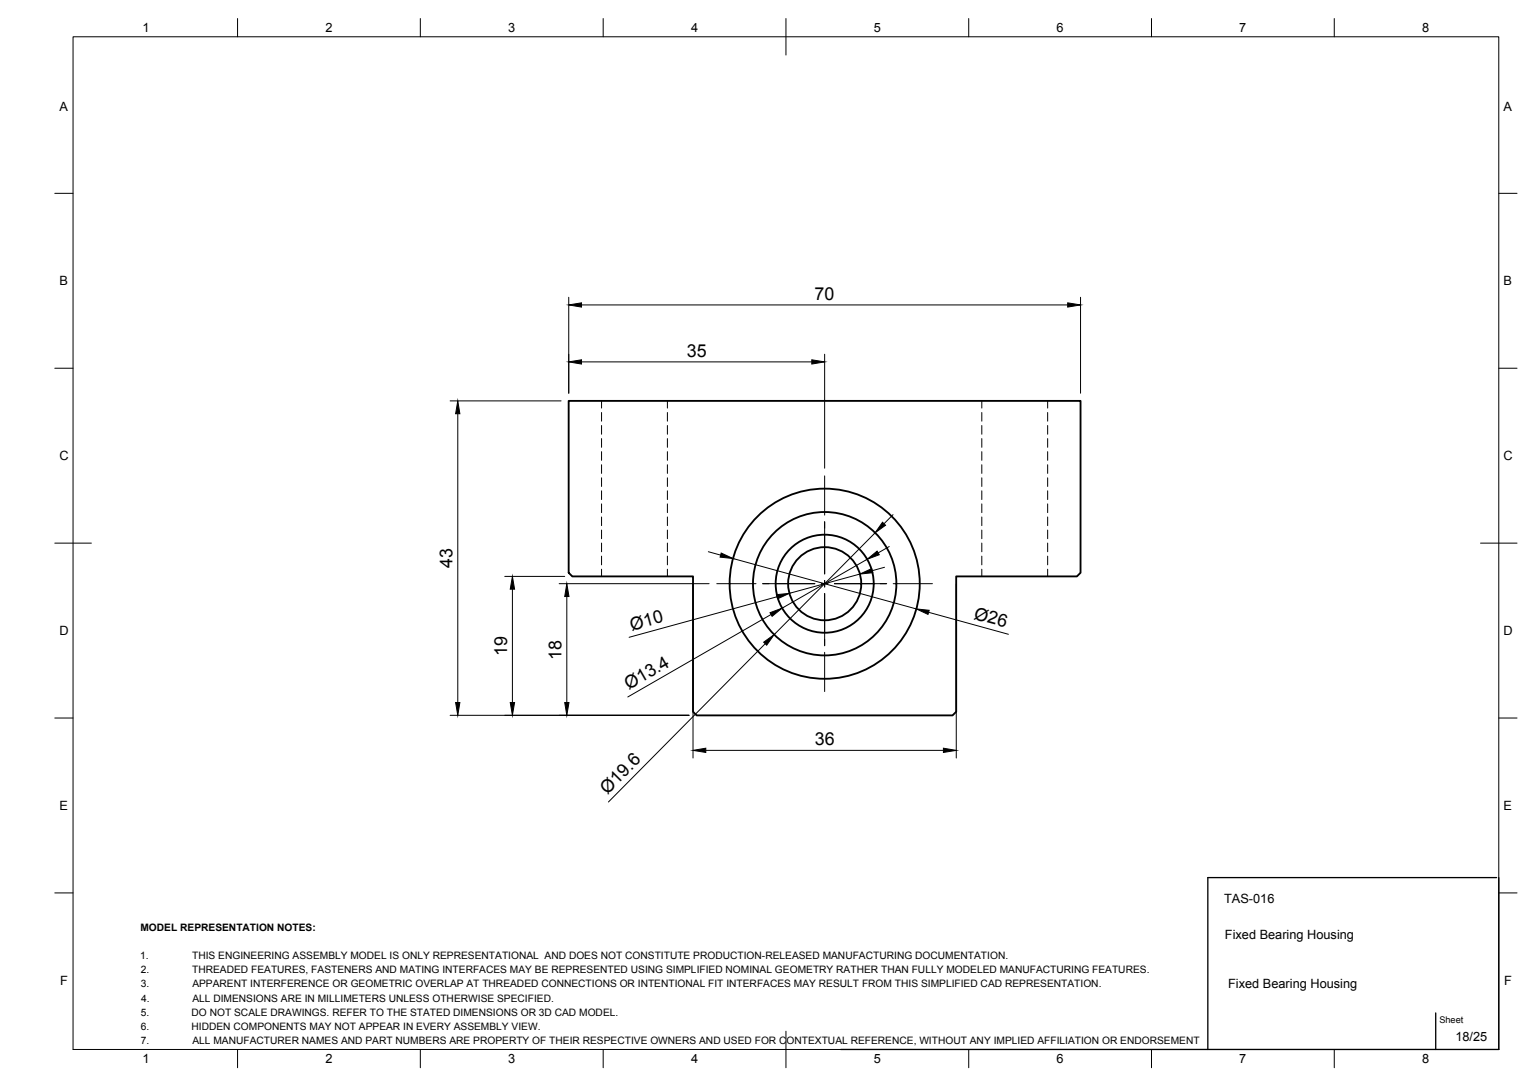
ISO-10303-21;
HEADER;
/* Generated by software containing ST-Developer
 * from STEP Tools, Inc. (www.steptools.com) 
 */

FILE_DESCRIPTION(
/* description */ ('STEP AP214'),
/* implementation_level */ '2;1');

FILE_NAME(
/* name */ 'Fixed Bearing Housing.step',
/* time_stamp */ '2026-11-15T14:55:55-08:00',
/* author */ (''),
/* organization */ (''),
/* preprocessor_version */ 'ST-DEVELOPER v20.2',
/* originating_system */ 'Autodesk Translation Framework v15.17.0.0',
/* authorisation */ '');

FILE_SCHEMA (('AUTOMOTIVE_DESIGN { 1 0 10303 214 3 1 1 }'));
ENDSEC;

DATA;
#10=MECHANICAL_DESIGN_GEOMETRIC_PRESENTATION_REPRESENTATION('',(#933,#934),#57079);
#644=TOROIDAL_SURFACE('',#25301,5.3,0.300000000000002);
#645=TOROIDAL_SURFACE('',#25307,5.3,0.300000000000002);
#646=TOROIDAL_SURFACE('',#25316,12.7,0.300000000000001);
#647=TOROIDAL_SURFACE('',#25322,12.7,0.300000000000002);
#874=SHAPE_REPRESENTATION_RELATIONSHIP('SRR','None',#57260,#903);
#903=ADVANCED_BREP_SHAPE_REPRESENTATION('',(#970,#971),#57052);
#933=STYLED_ITEM('',(#57444),#970);
#934=STYLED_ITEM('',(#57444),#971);
#970=MANIFOLD_SOLID_BREP('Body1',#24533);
#971=MANIFOLD_SOLID_BREP('Body2',#24534);
#1077=FACE_BOUND('',#3829,.T.);
#1078=FACE_BOUND('',#3831,.T.);
#1079=FACE_BOUND('',#3833,.T.);
#1080=FACE_BOUND('',#3837,.T.);
#1081=FACE_BOUND('',#3838,.T.);
#1082=FACE_BOUND('',#3842,.T.);
#1083=FACE_BOUND('',#3859,.T.);
#1084=FACE_BOUND('',#3861,.T.);
#1085=FACE_BOUND('',#3863,.T.);
#1086=FACE_BOUND('',#3865,.T.);
#1087=FACE_BOUND('',#3867,.T.);
#1088=FACE_BOUND('',#3869,.T.);
#1472=PLANE('',#25287);
#1473=PLANE('',#25288);
#1474=PLANE('',#25289);
#1475=PLANE('',#25290);
#1476=PLANE('',#25291);
#1477=PLANE('',#25292);
#1478=PLANE('',#25293);
#1479=PLANE('',#25294);
#1480=PLANE('',#25295);
#1481=PLANE('',#25296);
#1482=PLANE('',#25297);
#1483=PLANE('',#25298);
#1484=PLANE('',#25299);
#1485=PLANE('',#25300);
#1486=PLANE('',#25331);
#1487=PLANE('',#25332);
#1488=PLANE('',#25333);
#1489=PLANE('',#25334);
#1490=PLANE('',#25335);
#1491=PLANE('',#25336);
#2373=FACE_OUTER_BOUND('',#3825,.T.);
#2374=FACE_OUTER_BOUND('',#3826,.T.);
#2375=FACE_OUTER_BOUND('',#3827,.T.);
#2376=FACE_OUTER_BOUND('',#3828,.T.);
#2377=FACE_OUTER_BOUND('',#3830,.T.);
#2378=FACE_OUTER_BOUND('',#3832,.T.);
#2379=FACE_OUTER_BOUND('',#3834,.T.);
#2380=FACE_OUTER_BOUND('',#3835,.T.);
#2381=FACE_OUTER_BOUND('',#3836,.T.);
#2382=FACE_OUTER_BOUND('',#3839,.T.);
#2383=FACE_OUTER_BOUND('',#3840,.T.);
#2384=FACE_OUTER_BOUND('',#3841,.T.);
#2385=FACE_OUTER_BOUND('',#3843,.T.);
#2386=FACE_OUTER_BOUND('',#3844,.T.);
#2387=FACE_OUTER_BOUND('',#3845,.T.);
#2388=FACE_OUTER_BOUND('',#3846,.T.);
#2389=FACE_OUTER_BOUND('',#3847,.T.);
#2390=FACE_OUTER_BOUND('',#3848,.T.);
#2391=FACE_OUTER_BOUND('',#3849,.T.);
#2392=FACE_OUTER_BOUND('',#3850,.T.);
#2393=FACE_OUTER_BOUND('',#3851,.T.);
#2394=FACE_OUTER_BOUND('',#3852,.T.);
#2395=FACE_OUTER_BOUND('',#3853,.T.);
#2396=FACE_OUTER_BOUND('',#3854,.T.);
#2397=FACE_OUTER_BOUND('',#3855,.T.);
#2398=FACE_OUTER_BOUND('',#3856,.T.);
#2399=FACE_OUTER_BOUND('',#3857,.T.);
#2400=FACE_OUTER_BOUND('',#3858,.T.);
#2401=FACE_OUTER_BOUND('',#3860,.T.);
#2402=FACE_OUTER_BOUND('',#3862,.T.);
#2403=FACE_OUTER_BOUND('',#3864,.T.);
#2404=FACE_OUTER_BOUND('',#3866,.T.);
#2405=FACE_OUTER_BOUND('',#3868,.T.);
#3825=EDGE_LOOP('',(#16870,#16871,#16872,#16873));
#3826=EDGE_LOOP('',(#16874,#16875,#16876,#16877));
#3827=EDGE_LOOP('',(#16878,#16879,#16880,#16881));
#3828=EDGE_LOOP('',(#16882,#16883,#16884,#16885,#16886,#16887,#16888,#16889,
#16890,#16891,#16892,#16893));
#3829=EDGE_LOOP('',(#16894));
#3830=EDGE_LOOP('',(#16895,#16896,#16897,#16898,#16899,#16900,#16901,#16902,
#16903,#16904,#16905,#16906));
#3831=EDGE_LOOP('',(#16907));
#3832=EDGE_LOOP('',(#16908,#16909,#16910,#16911));
#3833=EDGE_LOOP('',(#16912));
#3834=EDGE_LOOP('',(#16913,#16914,#16915,#16916));
#3835=EDGE_LOOP('',(#16917,#16918,#16919,#16920));
#3836=EDGE_LOOP('',(#16921,#16922,#16923,#16924));
#3837=EDGE_LOOP('',(#16925));
#3838=EDGE_LOOP('',(#16926));
#3839=EDGE_LOOP('',(#16927,#16928,#16929,#16930));
#3840=EDGE_LOOP('',(#16931,#16932,#16933,#16934));
#3841=EDGE_LOOP('',(#16935,#16936,#16937,#16938));
#3842=EDGE_LOOP('',(#16939));
#3843=EDGE_LOOP('',(#16940,#16941,#16942,#16943));
#3844=EDGE_LOOP('',(#16944,#16945,#16946,#16947));
#3845=EDGE_LOOP('',(#16948,#16949,#16950,#16951));
#3846=EDGE_LOOP('',(#16952,#16953,#16954,#16955));
#3847=EDGE_LOOP('',(#16956,#16957,#16958,#16959));
#3848=EDGE_LOOP('',(#16960,#16961,#16962,#16963));
#3849=EDGE_LOOP('',(#16964,#16965,#16966,#16967));
#3850=EDGE_LOOP('',(#16968,#16969,#16970,#16971));
#3851=EDGE_LOOP('',(#16972,#16973,#16974,#16975));
#3852=EDGE_LOOP('',(#16976,#16977,#16978,#16979));
#3853=EDGE_LOOP('',(#16980,#16981,#16982,#16983));
#3854=EDGE_LOOP('',(#16984,#16985,#16986,#16987));
#3855=EDGE_LOOP('',(#16988,#16989,#16990,#16991));
#3856=EDGE_LOOP('',(#16992,#16993,#16994,#16995));
#3857=EDGE_LOOP('',(#16996,#16997,#16998,#16999));
#3858=EDGE_LOOP('',(#17000));
#3859=EDGE_LOOP('',(#17001));
#3860=EDGE_LOOP('',(#17002));
#3861=EDGE_LOOP('',(#17003));
#3862=EDGE_LOOP('',(#17004));
#3863=EDGE_LOOP('',(#17005));
#3864=EDGE_LOOP('',(#17006));
#3865=EDGE_LOOP('',(#17007));
#3866=EDGE_LOOP('',(#17008));
#3867=EDGE_LOOP('',(#17009));
#3868=EDGE_LOOP('',(#17010));
#3869=EDGE_LOOP('',(#17011));
#5550=LINE('',#35882,#7517);
#5551=LINE('',#35888,#7518);
#5552=LINE('',#35894,#7519);
#5553=LINE('',#35899,#7520);
#5554=LINE('',#35901,#7521);
#5555=LINE('',#35903,#7522);
#5556=LINE('',#35905,#7523);
#5557=LINE('',#35907,#7524);
#5558=LINE('',#35909,#7525);
#5559=LINE('',#35911,#7526);
#5560=LINE('',#35913,#7527);
#5561=LINE('',#35915,#7528);
#5562=LINE('',#35917,#7529);
#5563=LINE('',#35919,#7530);
#5564=LINE('',#35920,#7531);
#5565=LINE('',#35924,#7532);
#5566=LINE('',#35926,#7533);
#5567=LINE('',#35928,#7534);
#5568=LINE('',#35930,#7535);
#5569=LINE('',#35932,#7536);
#5570=LINE('',#35934,#7537);
#5571=LINE('',#35936,#7538);
#5572=LINE('',#35938,#7539);
#5573=LINE('',#35940,#7540);
#5574=LINE('',#35942,#7541);
#5575=LINE('',#35944,#7542);
#5576=LINE('',#35945,#7543);
#5577=LINE('',#35947,#7544);
#5578=LINE('',#35948,#7545);
#5579=LINE('',#35950,#7546);
#5580=LINE('',#35952,#7547);
#5581=LINE('',#35954,#7548);
#5582=LINE('',#35956,#7549);
#5583=LINE('',#35958,#7550);
#5584=LINE('',#35960,#7551);
#5585=LINE('',#35962,#7552);
#5586=LINE('',#35964,#7553);
#5587=LINE('',#35966,#7554);
#5588=LINE('',#35968,#7555);
#5589=LINE('',#35978,#7556);
#5590=LINE('',#35988,#7557);
#5591=LINE('',#35994,#7558);
#5592=LINE('',#36004,#7559);
#5593=LINE('',#36014,#7560);
#5594=LINE('',#36020,#7561);
#7517=VECTOR('',#28570,4.49999999999999);
#7518=VECTOR('',#28577,4.49999999999999);
#7519=VECTOR('',#28584,13.);
#7520=VECTOR('',#28589,1000.);
#7521=VECTOR('',#28590,1000.);
#7522=VECTOR('',#28591,1000.);
#7523=VECTOR('',#28592,1000.);
#7524=VECTOR('',#28593,1000.);
#7525=VECTOR('',#28594,1000.);
#7526=VECTOR('',#28595,1000.);
#7527=VECTOR('',#28596,1000.);
#7528=VECTOR('',#28597,1000.);
#7529=VECTOR('',#28598,1000.);
#7530=VECTOR('',#28599,1000.);
#7531=VECTOR('',#28600,1000.);
#7532=VECTOR('',#28603,1000.);
#7533=VECTOR('',#28604,1000.);
#7534=VECTOR('',#28605,1000.);
#7535=VECTOR('',#28606,1000.);
#7536=VECTOR('',#28607,1000.);
#7537=VECTOR('',#28608,1000.);
#7538=VECTOR('',#28609,1000.);
#7539=VECTOR('',#28610,1000.);
#7540=VECTOR('',#28611,1000.);
#7541=VECTOR('',#28612,1000.);
#7542=VECTOR('',#28613,1000.);
#7543=VECTOR('',#28614,1000.);
#7544=VECTOR('',#28617,1000.);
#7545=VECTOR('',#28618,1000.);
#7546=VECTOR('',#28621,1000.);
#7547=VECTOR('',#28624,1000.);
#7548=VECTOR('',#28627,1000.);
#7549=VECTOR('',#28630,1000.);
#7550=VECTOR('',#28633,1000.);
#7551=VECTOR('',#28636,1000.);
#7552=VECTOR('',#28639,1000.);
#7553=VECTOR('',#28642,1000.);
#7554=VECTOR('',#28645,1000.);
#7555=VECTOR('',#28648,1000.);
#7556=VECTOR('',#28661,5.);
#7557=VECTOR('',#28674,6.7);
#7558=VECTOR('',#28681,9.8);
#7559=VECTOR('',#28694,13.);
#7560=VECTOR('',#28707,9.8);
#7561=VECTOR('',#28714,6.69999999999999);
#9348=CIRCLE('',#25279,4.5);
#9349=CIRCLE('',#25280,4.49999999999999);
#9350=CIRCLE('',#25282,4.5);
#9351=CIRCLE('',#25283,4.49999999999999);
#9352=CIRCLE('',#25285,13.);
#9353=CIRCLE('',#25286,13.);
#9354=CIRCLE('',#25302,5.3);
#9355=CIRCLE('',#25303,0.300000000000002);
#9356=CIRCLE('',#25304,4.99999999999999);
#9357=CIRCLE('',#25306,5.);
#9358=CIRCLE('',#25308,0.300000000000002);
#9359=CIRCLE('',#25309,5.3);
#9360=CIRCLE('',#25311,6.7);
#9361=CIRCLE('',#25312,6.7);
#9362=CIRCLE('',#25314,9.8);
#9363=CIRCLE('',#25315,9.8);
#9364=CIRCLE('',#25317,12.7);
#9365=CIRCLE('',#25318,0.300000000000001);
#9366=CIRCLE('',#25319,13.);
#9367=CIRCLE('',#25321,13.);
#9368=CIRCLE('',#25323,0.300000000000002);
#9369=CIRCLE('',#25324,12.7);
#9370=CIRCLE('',#25326,9.8);
#9371=CIRCLE('',#25327,9.8);
#9372=CIRCLE('',#25329,6.69999999999999);
#9373=CIRCLE('',#25330,6.69999999999999);
#10589=VERTEX_POINT('',#35879);
#10590=VERTEX_POINT('',#35881);
#10591=VERTEX_POINT('',#35885);
#10592=VERTEX_POINT('',#35887);
#10593=VERTEX_POINT('',#35891);
#10594=VERTEX_POINT('',#35893);
#10595=VERTEX_POINT('',#35897);
#10596=VERTEX_POINT('',#35898);
#10597=VERTEX_POINT('',#35900);
#10598=VERTEX_POINT('',#35902);
#10599=VERTEX_POINT('',#35904);
#10600=VERTEX_POINT('',#35906);
#10601=VERTEX_POINT('',#35908);
#10602=VERTEX_POINT('',#35910);
#10603=VERTEX_POINT('',#35912);
#10604=VERTEX_POINT('',#35914);
#10605=VERTEX_POINT('',#35916);
#10606=VERTEX_POINT('',#35918);
#10607=VERTEX_POINT('',#35922);
#10608=VERTEX_POINT('',#35923);
#10609=VERTEX_POINT('',#35925);
#10610=VERTEX_POINT('',#35927);
#10611=VERTEX_POINT('',#35929);
#10612=VERTEX_POINT('',#35931);
#10613=VERTEX_POINT('',#35933);
#10614=VERTEX_POINT('',#35935);
#10615=VERTEX_POINT('',#35937);
#10616=VERTEX_POINT('',#35939);
#10617=VERTEX_POINT('',#35941);
#10618=VERTEX_POINT('',#35943);
#10619=VERTEX_POINT('',#35971);
#10620=VERTEX_POINT('',#35973);
#10621=VERTEX_POINT('',#35977);
#10622=VERTEX_POINT('',#35981);
#10623=VERTEX_POINT('',#35985);
#10624=VERTEX_POINT('',#35987);
#10625=VERTEX_POINT('',#35991);
#10626=VERTEX_POINT('',#35993);
#10627=VERTEX_POINT('',#35997);
#10628=VERTEX_POINT('',#35999);
#10629=VERTEX_POINT('',#36003);
#10630=VERTEX_POINT('',#36007);
#10631=VERTEX_POINT('',#36011);
#10632=VERTEX_POINT('',#36013);
#10633=VERTEX_POINT('',#36017);
#10634=VERTEX_POINT('',#36019);
#12980=EDGE_CURVE('',#10589,#10589,#9348,.T.);
#12981=EDGE_CURVE('',#10589,#10590,#5550,.T.);
#12982=EDGE_CURVE('',#10590,#10590,#9349,.T.);
#12983=EDGE_CURVE('',#10591,#10591,#9350,.T.);
#12984=EDGE_CURVE('',#10591,#10592,#5551,.T.);
#12985=EDGE_CURVE('',#10592,#10592,#9351,.T.);
#12986=EDGE_CURVE('',#10593,#10593,#9352,.T.);
#12987=EDGE_CURVE('',#10593,#10594,#5552,.T.);
#12988=EDGE_CURVE('',#10594,#10594,#9353,.T.);
#12989=EDGE_CURVE('',#10595,#10596,#5553,.T.);
#12990=EDGE_CURVE('',#10596,#10597,#5554,.T.);
#12991=EDGE_CURVE('',#10597,#10598,#5555,.T.);
#12992=EDGE_CURVE('',#10598,#10599,#5556,.T.);
#12993=EDGE_CURVE('',#10599,#10600,#5557,.T.);
#12994=EDGE_CURVE('',#10600,#10601,#5558,.T.);
#12995=EDGE_CURVE('',#10601,#10602,#5559,.T.);
#12996=EDGE_CURVE('',#10602,#10603,#5560,.T.);
#12997=EDGE_CURVE('',#10603,#10604,#5561,.T.);
#12998=EDGE_CURVE('',#10604,#10605,#5562,.T.);
#12999=EDGE_CURVE('',#10605,#10606,#5563,.T.);
#13000=EDGE_CURVE('',#10606,#10595,#5564,.T.);
#13001=EDGE_CURVE('',#10607,#10608,#5565,.T.);
#13002=EDGE_CURVE('',#10609,#10607,#5566,.T.);
#13003=EDGE_CURVE('',#10610,#10609,#5567,.T.);
#13004=EDGE_CURVE('',#10611,#10610,#5568,.T.);
#13005=EDGE_CURVE('',#10612,#10611,#5569,.T.);
#13006=EDGE_CURVE('',#10613,#10612,#5570,.T.);
#13007=EDGE_CURVE('',#10614,#10613,#5571,.T.);
#13008=EDGE_CURVE('',#10615,#10614,#5572,.T.);
#13009=EDGE_CURVE('',#10616,#10615,#5573,.T.);
#13010=EDGE_CURVE('',#10617,#10616,#5574,.T.);
#13011=EDGE_CURVE('',#10618,#10617,#5575,.T.);
#13012=EDGE_CURVE('',#10608,#10618,#5576,.T.);
#13013=EDGE_CURVE('',#10596,#10608,#5577,.T.);
#13014=EDGE_CURVE('',#10595,#10607,#5578,.T.);
#13015=EDGE_CURVE('',#10597,#10618,#5579,.T.);
#13016=EDGE_CURVE('',#10598,#10617,#5580,.T.);
#13017=EDGE_CURVE('',#10599,#10616,#5581,.T.);
#13018=EDGE_CURVE('',#10600,#10615,#5582,.T.);
#13019=EDGE_CURVE('',#10601,#10614,#5583,.T.);
#13020=EDGE_CURVE('',#10602,#10613,#5584,.T.);
#13021=EDGE_CURVE('',#10603,#10612,#5585,.T.);
#13022=EDGE_CURVE('',#10604,#10611,#5586,.T.);
#13023=EDGE_CURVE('',#10605,#10610,#5587,.T.);
#13024=EDGE_CURVE('',#10606,#10609,#5588,.T.);
#13025=EDGE_CURVE('',#10619,#10619,#9354,.T.);
#13026=EDGE_CURVE('',#10619,#10620,#9355,.T.);
#13027=EDGE_CURVE('',#10620,#10620,#9356,.T.);
#13028=EDGE_CURVE('',#10620,#10621,#5589,.T.);
#13029=EDGE_CURVE('',#10621,#10621,#9357,.T.);
#13030=EDGE_CURVE('',#10621,#10622,#9358,.T.);
#13031=EDGE_CURVE('',#10622,#10622,#9359,.T.);
#13032=EDGE_CURVE('',#10623,#10623,#9360,.T.);
#13033=EDGE_CURVE('',#10623,#10624,#5590,.T.);
#13034=EDGE_CURVE('',#10624,#10624,#9361,.T.);
#13035=EDGE_CURVE('',#10625,#10625,#9362,.T.);
#13036=EDGE_CURVE('',#10625,#10626,#5591,.T.);
#13037=EDGE_CURVE('',#10626,#10626,#9363,.T.);
#13038=EDGE_CURVE('',#10627,#10627,#9364,.T.);
#13039=EDGE_CURVE('',#10627,#10628,#9365,.T.);
#13040=EDGE_CURVE('',#10628,#10628,#9366,.T.);
#13041=EDGE_CURVE('',#10628,#10629,#5592,.T.);
#13042=EDGE_CURVE('',#10629,#10629,#9367,.T.);
#13043=EDGE_CURVE('',#10629,#10630,#9368,.T.);
#13044=EDGE_CURVE('',#10630,#10630,#9369,.T.);
#13045=EDGE_CURVE('',#10631,#10631,#9370,.T.);
#13046=EDGE_CURVE('',#10631,#10632,#5593,.T.);
#13047=EDGE_CURVE('',#10632,#10632,#9371,.T.);
#13048=EDGE_CURVE('',#10633,#10633,#9372,.T.);
#13049=EDGE_CURVE('',#10633,#10634,#5594,.T.);
#13050=EDGE_CURVE('',#10634,#10634,#9373,.T.);
#16870=ORIENTED_EDGE('',*,*,#12980,.F.);
#16871=ORIENTED_EDGE('',*,*,#12981,.T.);
#16872=ORIENTED_EDGE('',*,*,#12982,.T.);
#16873=ORIENTED_EDGE('',*,*,#12981,.F.);
#16874=ORIENTED_EDGE('',*,*,#12983,.F.);
#16875=ORIENTED_EDGE('',*,*,#12984,.T.);
#16876=ORIENTED_EDGE('',*,*,#12985,.T.);
#16877=ORIENTED_EDGE('',*,*,#12984,.F.);
#16878=ORIENTED_EDGE('',*,*,#12986,.T.);
#16879=ORIENTED_EDGE('',*,*,#12987,.T.);
#16880=ORIENTED_EDGE('',*,*,#12988,.F.);
#16881=ORIENTED_EDGE('',*,*,#12987,.F.);
#16882=ORIENTED_EDGE('',*,*,#12989,.T.);
#16883=ORIENTED_EDGE('',*,*,#12990,.T.);
#16884=ORIENTED_EDGE('',*,*,#12991,.T.);
#16885=ORIENTED_EDGE('',*,*,#12992,.T.);
#16886=ORIENTED_EDGE('',*,*,#12993,.T.);
#16887=ORIENTED_EDGE('',*,*,#12994,.T.);
#16888=ORIENTED_EDGE('',*,*,#12995,.T.);
#16889=ORIENTED_EDGE('',*,*,#12996,.T.);
#16890=ORIENTED_EDGE('',*,*,#12997,.T.);
#16891=ORIENTED_EDGE('',*,*,#12998,.T.);
#16892=ORIENTED_EDGE('',*,*,#12999,.T.);
#16893=ORIENTED_EDGE('',*,*,#13000,.T.);
#16894=ORIENTED_EDGE('',*,*,#12986,.F.);
#16895=ORIENTED_EDGE('',*,*,#13001,.F.);
#16896=ORIENTED_EDGE('',*,*,#13002,.F.);
#16897=ORIENTED_EDGE('',*,*,#13003,.F.);
#16898=ORIENTED_EDGE('',*,*,#13004,.F.);
#16899=ORIENTED_EDGE('',*,*,#13005,.F.);
#16900=ORIENTED_EDGE('',*,*,#13006,.F.);
#16901=ORIENTED_EDGE('',*,*,#13007,.F.);
#16902=ORIENTED_EDGE('',*,*,#13008,.F.);
#16903=ORIENTED_EDGE('',*,*,#13009,.F.);
#16904=ORIENTED_EDGE('',*,*,#13010,.F.);
#16905=ORIENTED_EDGE('',*,*,#13011,.F.);
#16906=ORIENTED_EDGE('',*,*,#13012,.F.);
#16907=ORIENTED_EDGE('',*,*,#12988,.T.);
#16908=ORIENTED_EDGE('',*,*,#13001,.T.);
#16909=ORIENTED_EDGE('',*,*,#13013,.F.);
#16910=ORIENTED_EDGE('',*,*,#12989,.F.);
#16911=ORIENTED_EDGE('',*,*,#13014,.T.);
#16912=ORIENTED_EDGE('',*,*,#12982,.F.);
#16913=ORIENTED_EDGE('',*,*,#13012,.T.);
#16914=ORIENTED_EDGE('',*,*,#13015,.F.);
#16915=ORIENTED_EDGE('',*,*,#12990,.F.);
#16916=ORIENTED_EDGE('',*,*,#13013,.T.);
#16917=ORIENTED_EDGE('',*,*,#13011,.T.);
#16918=ORIENTED_EDGE('',*,*,#13016,.F.);
#16919=ORIENTED_EDGE('',*,*,#12991,.F.);
#16920=ORIENTED_EDGE('',*,*,#13015,.T.);
#16921=ORIENTED_EDGE('',*,*,#13010,.T.);
#16922=ORIENTED_EDGE('',*,*,#13017,.F.);
#16923=ORIENTED_EDGE('',*,*,#12992,.F.);
#16924=ORIENTED_EDGE('',*,*,#13016,.T.);
#16925=ORIENTED_EDGE('',*,*,#12980,.T.);
#16926=ORIENTED_EDGE('',*,*,#12983,.T.);
#16927=ORIENTED_EDGE('',*,*,#13009,.T.);
#16928=ORIENTED_EDGE('',*,*,#13018,.F.);
#16929=ORIENTED_EDGE('',*,*,#12993,.F.);
#16930=ORIENTED_EDGE('',*,*,#13017,.T.);
#16931=ORIENTED_EDGE('',*,*,#13008,.T.);
#16932=ORIENTED_EDGE('',*,*,#13019,.F.);
#16933=ORIENTED_EDGE('',*,*,#12994,.F.);
#16934=ORIENTED_EDGE('',*,*,#13018,.T.);
#16935=ORIENTED_EDGE('',*,*,#13007,.T.);
#16936=ORIENTED_EDGE('',*,*,#13020,.F.);
#16937=ORIENTED_EDGE('',*,*,#12995,.F.);
#16938=ORIENTED_EDGE('',*,*,#13019,.T.);
#16939=ORIENTED_EDGE('',*,*,#12985,.F.);
#16940=ORIENTED_EDGE('',*,*,#13006,.T.);
#16941=ORIENTED_EDGE('',*,*,#13021,.F.);
#16942=ORIENTED_EDGE('',*,*,#12996,.F.);
#16943=ORIENTED_EDGE('',*,*,#13020,.T.);
#16944=ORIENTED_EDGE('',*,*,#13005,.T.);
#16945=ORIENTED_EDGE('',*,*,#13022,.F.);
#16946=ORIENTED_EDGE('',*,*,#12997,.F.);
#16947=ORIENTED_EDGE('',*,*,#13021,.T.);
#16948=ORIENTED_EDGE('',*,*,#13004,.T.);
#16949=ORIENTED_EDGE('',*,*,#13023,.F.);
#16950=ORIENTED_EDGE('',*,*,#12998,.F.);
#16951=ORIENTED_EDGE('',*,*,#13022,.T.);
#16952=ORIENTED_EDGE('',*,*,#13003,.T.);
#16953=ORIENTED_EDGE('',*,*,#13024,.F.);
#16954=ORIENTED_EDGE('',*,*,#12999,.F.);
#16955=ORIENTED_EDGE('',*,*,#13023,.T.);
#16956=ORIENTED_EDGE('',*,*,#13002,.T.);
#16957=ORIENTED_EDGE('',*,*,#13014,.F.);
#16958=ORIENTED_EDGE('',*,*,#13000,.F.);
#16959=ORIENTED_EDGE('',*,*,#13024,.T.);
#16960=ORIENTED_EDGE('',*,*,#13025,.F.);
#16961=ORIENTED_EDGE('',*,*,#13026,.T.);
#16962=ORIENTED_EDGE('',*,*,#13027,.T.);
#16963=ORIENTED_EDGE('',*,*,#13026,.F.);
#16964=ORIENTED_EDGE('',*,*,#13027,.F.);
#16965=ORIENTED_EDGE('',*,*,#13028,.T.);
#16966=ORIENTED_EDGE('',*,*,#13029,.T.);
#16967=ORIENTED_EDGE('',*,*,#13028,.F.);
#16968=ORIENTED_EDGE('',*,*,#13029,.F.);
#16969=ORIENTED_EDGE('',*,*,#13030,.T.);
#16970=ORIENTED_EDGE('',*,*,#13031,.T.);
#16971=ORIENTED_EDGE('',*,*,#13030,.F.);
#16972=ORIENTED_EDGE('',*,*,#13032,.F.);
#16973=ORIENTED_EDGE('',*,*,#13033,.T.);
#16974=ORIENTED_EDGE('',*,*,#13034,.T.);
#16975=ORIENTED_EDGE('',*,*,#13033,.F.);
#16976=ORIENTED_EDGE('',*,*,#13035,.F.);
#16977=ORIENTED_EDGE('',*,*,#13036,.T.);
#16978=ORIENTED_EDGE('',*,*,#13037,.T.);
#16979=ORIENTED_EDGE('',*,*,#13036,.F.);
#16980=ORIENTED_EDGE('',*,*,#13038,.F.);
#16981=ORIENTED_EDGE('',*,*,#13039,.T.);
#16982=ORIENTED_EDGE('',*,*,#13040,.T.);
#16983=ORIENTED_EDGE('',*,*,#13039,.F.);
#16984=ORIENTED_EDGE('',*,*,#13040,.F.);
#16985=ORIENTED_EDGE('',*,*,#13041,.T.);
#16986=ORIENTED_EDGE('',*,*,#13042,.T.);
#16987=ORIENTED_EDGE('',*,*,#13041,.F.);
#16988=ORIENTED_EDGE('',*,*,#13042,.F.);
#16989=ORIENTED_EDGE('',*,*,#13043,.T.);
#16990=ORIENTED_EDGE('',*,*,#13044,.T.);
#16991=ORIENTED_EDGE('',*,*,#13043,.F.);
#16992=ORIENTED_EDGE('',*,*,#13045,.F.);
#16993=ORIENTED_EDGE('',*,*,#13046,.T.);
#16994=ORIENTED_EDGE('',*,*,#13047,.T.);
#16995=ORIENTED_EDGE('',*,*,#13046,.F.);
#16996=ORIENTED_EDGE('',*,*,#13048,.F.);
#16997=ORIENTED_EDGE('',*,*,#13049,.T.);
#16998=ORIENTED_EDGE('',*,*,#13050,.T.);
#16999=ORIENTED_EDGE('',*,*,#13049,.F.);
#17000=ORIENTED_EDGE('',*,*,#13047,.F.);
#17001=ORIENTED_EDGE('',*,*,#13048,.T.);
#17002=ORIENTED_EDGE('',*,*,#13044,.F.);
#17003=ORIENTED_EDGE('',*,*,#13045,.T.);
#17004=ORIENTED_EDGE('',*,*,#13038,.T.);
#17005=ORIENTED_EDGE('',*,*,#13037,.F.);
#17006=ORIENTED_EDGE('',*,*,#13035,.T.);
#17007=ORIENTED_EDGE('',*,*,#13034,.F.);
#17008=ORIENTED_EDGE('',*,*,#13032,.T.);
#17009=ORIENTED_EDGE('',*,*,#13031,.F.);
#17010=ORIENTED_EDGE('',*,*,#13050,.F.);
#17011=ORIENTED_EDGE('',*,*,#13025,.T.);
#22801=CYLINDRICAL_SURFACE('',#25278,4.49999999999999);
#22802=CYLINDRICAL_SURFACE('',#25281,4.49999999999999);
#22803=CYLINDRICAL_SURFACE('',#25284,13.);
#22804=CYLINDRICAL_SURFACE('',#25305,5.);
#22805=CYLINDRICAL_SURFACE('',#25310,6.7);
#22806=CYLINDRICAL_SURFACE('',#25313,9.8);
#22807=CYLINDRICAL_SURFACE('',#25320,13.);
#22808=CYLINDRICAL_SURFACE('',#25325,9.8);
#22809=CYLINDRICAL_SURFACE('',#25328,6.69999999999999);
#23365=ADVANCED_FACE('',(#2373),#22801,.F.);
#23366=ADVANCED_FACE('',(#2374),#22802,.F.);
#23367=ADVANCED_FACE('',(#2375),#22803,.F.);
#23368=ADVANCED_FACE('',(#2376,#1077),#1472,.T.);
#23369=ADVANCED_FACE('',(#2377,#1078),#1473,.F.);
#23370=ADVANCED_FACE('',(#2378,#1079),#1474,.F.);
#23371=ADVANCED_FACE('',(#2379),#1475,.F.);
#23372=ADVANCED_FACE('',(#2380),#1476,.F.);
#23373=ADVANCED_FACE('',(#2381,#1080,#1081),#1477,.F.);
#23374=ADVANCED_FACE('',(#2382),#1478,.F.);
#23375=ADVANCED_FACE('',(#2383),#1479,.F.);
#23376=ADVANCED_FACE('',(#2384,#1082),#1480,.F.);
#23377=ADVANCED_FACE('',(#2385),#1481,.F.);
#23378=ADVANCED_FACE('',(#2386),#1482,.F.);
#23379=ADVANCED_FACE('',(#2387),#1483,.F.);
#23380=ADVANCED_FACE('',(#2388),#1484,.F.);
#23381=ADVANCED_FACE('',(#2389),#1485,.F.);
#23382=ADVANCED_FACE('',(#2390),#644,.T.);
#23383=ADVANCED_FACE('',(#2391),#22804,.F.);
#23384=ADVANCED_FACE('',(#2392),#645,.T.);
#23385=ADVANCED_FACE('',(#2393),#22805,.T.);
#23386=ADVANCED_FACE('',(#2394),#22806,.F.);
#23387=ADVANCED_FACE('',(#2395),#646,.T.);
#23388=ADVANCED_FACE('',(#2396),#22807,.T.);
#23389=ADVANCED_FACE('',(#2397),#647,.T.);
#23390=ADVANCED_FACE('',(#2398),#22808,.F.);
#23391=ADVANCED_FACE('',(#2399),#22809,.T.);
#23392=ADVANCED_FACE('',(#2400,#1083),#1486,.F.);
#23393=ADVANCED_FACE('',(#2401,#1084),#1487,.F.);
#23394=ADVANCED_FACE('',(#2402,#1085),#1488,.F.);
#23395=ADVANCED_FACE('',(#2403,#1086),#1489,.F.);
#23396=ADVANCED_FACE('',(#2404,#1087),#1490,.F.);
#23397=ADVANCED_FACE('',(#2405,#1088),#1491,.F.);
#24533=CLOSED_SHELL('',(#23365,#23366,#23367,#23368,#23369,#23370,#23371,
#23372,#23373,#23374,#23375,#23376,#23377,#23378,#23379,#23380,#23381));
#24534=CLOSED_SHELL('',(#23382,#23383,#23384,#23385,#23386,#23387,#23388,
#23389,#23390,#23391,#23392,#23393,#23394,#23395,#23396,#23397));
#25277=AXIS2_PLACEMENT_3D('',#35877,#28564,#28565);
#25278=AXIS2_PLACEMENT_3D('',#35878,#28566,#28567);
#25279=AXIS2_PLACEMENT_3D('',#35880,#28568,#28569);
#25280=AXIS2_PLACEMENT_3D('',#35883,#28571,#28572);
#25281=AXIS2_PLACEMENT_3D('',#35884,#28573,#28574);
#25282=AXIS2_PLACEMENT_3D('',#35886,#28575,#28576);
#25283=AXIS2_PLACEMENT_3D('',#35889,#28578,#28579);
#25284=AXIS2_PLACEMENT_3D('',#35890,#28580,#28581);
#25285=AXIS2_PLACEMENT_3D('',#35892,#28582,#28583);
#25286=AXIS2_PLACEMENT_3D('',#35895,#28585,#28586);
#25287=AXIS2_PLACEMENT_3D('',#35896,#28587,#28588);
#25288=AXIS2_PLACEMENT_3D('',#35921,#28601,#28602);
#25289=AXIS2_PLACEMENT_3D('',#35946,#28615,#28616);
#25290=AXIS2_PLACEMENT_3D('',#35949,#28619,#28620);
#25291=AXIS2_PLACEMENT_3D('',#35951,#28622,#28623);
#25292=AXIS2_PLACEMENT_3D('',#35953,#28625,#28626);
#25293=AXIS2_PLACEMENT_3D('',#35955,#28628,#28629);
#25294=AXIS2_PLACEMENT_3D('',#35957,#28631,#28632);
#25295=AXIS2_PLACEMENT_3D('',#35959,#28634,#28635);
#25296=AXIS2_PLACEMENT_3D('',#35961,#28637,#28638);
#25297=AXIS2_PLACEMENT_3D('',#35963,#28640,#28641);
#25298=AXIS2_PLACEMENT_3D('',#35965,#28643,#28644);
#25299=AXIS2_PLACEMENT_3D('',#35967,#28646,#28647);
#25300=AXIS2_PLACEMENT_3D('',#35969,#28649,#28650);
#25301=AXIS2_PLACEMENT_3D('',#35970,#28651,#28652);
#25302=AXIS2_PLACEMENT_3D('',#35972,#28653,#28654);
#25303=AXIS2_PLACEMENT_3D('',#35974,#28655,#28656);
#25304=AXIS2_PLACEMENT_3D('',#35975,#28657,#28658);
#25305=AXIS2_PLACEMENT_3D('',#35976,#28659,#28660);
#25306=AXIS2_PLACEMENT_3D('',#35979,#28662,#28663);
#25307=AXIS2_PLACEMENT_3D('',#35980,#28664,#28665);
#25308=AXIS2_PLACEMENT_3D('',#35982,#28666,#28667);
#25309=AXIS2_PLACEMENT_3D('',#35983,#28668,#28669);
#25310=AXIS2_PLACEMENT_3D('',#35984,#28670,#28671);
#25311=AXIS2_PLACEMENT_3D('',#35986,#28672,#28673);
#25312=AXIS2_PLACEMENT_3D('',#35989,#28675,#28676);
#25313=AXIS2_PLACEMENT_3D('',#35990,#28677,#28678);
#25314=AXIS2_PLACEMENT_3D('',#35992,#28679,#28680);
#25315=AXIS2_PLACEMENT_3D('',#35995,#28682,#28683);
#25316=AXIS2_PLACEMENT_3D('',#35996,#28684,#28685);
#25317=AXIS2_PLACEMENT_3D('',#35998,#28686,#28687);
#25318=AXIS2_PLACEMENT_3D('',#36000,#28688,#28689);
#25319=AXIS2_PLACEMENT_3D('',#36001,#28690,#28691);
#25320=AXIS2_PLACEMENT_3D('',#36002,#28692,#28693);
#25321=AXIS2_PLACEMENT_3D('',#36005,#28695,#28696);
#25322=AXIS2_PLACEMENT_3D('',#36006,#28697,#28698);
#25323=AXIS2_PLACEMENT_3D('',#36008,#28699,#28700);
#25324=AXIS2_PLACEMENT_3D('',#36009,#28701,#28702);
#25325=AXIS2_PLACEMENT_3D('',#36010,#28703,#28704);
#25326=AXIS2_PLACEMENT_3D('',#36012,#28705,#28706);
#25327=AXIS2_PLACEMENT_3D('',#36015,#28708,#28709);
#25328=AXIS2_PLACEMENT_3D('',#36016,#28710,#28711);
#25329=AXIS2_PLACEMENT_3D('',#36018,#28712,#28713);
#25330=AXIS2_PLACEMENT_3D('',#36021,#28715,#28716);
#25331=AXIS2_PLACEMENT_3D('',#36022,#28717,#28718);
#25332=AXIS2_PLACEMENT_3D('',#36023,#28719,#28720);
#25333=AXIS2_PLACEMENT_3D('',#36024,#28721,#28722);
#25334=AXIS2_PLACEMENT_3D('',#36025,#28723,#28724);
#25335=AXIS2_PLACEMENT_3D('',#36026,#28725,#28726);
#25336=AXIS2_PLACEMENT_3D('',#36027,#28727,#28728);
#28564=DIRECTION('axis',(0.,0.,1.));
#28565=DIRECTION('refdir',(1.,0.,0.));
#28566=DIRECTION('center_axis',(0.,1.,3.01691039300315E-16));
#28567=DIRECTION('ref_axis',(0.,-3.01691039300315E-16,1.));
#28568=DIRECTION('center_axis',(0.,1.,3.01691039300315E-16));
#28569=DIRECTION('ref_axis',(0.,-3.01691039300315E-16,1.));
#28570=DIRECTION('',(0.,1.,3.01691039300315E-16));
#28571=DIRECTION('center_axis',(0.,1.,3.01691039300315E-16));
#28572=DIRECTION('ref_axis',(0.,-3.01691039300315E-16,1.));
#28573=DIRECTION('center_axis',(0.,1.,3.01691039300315E-16));
#28574=DIRECTION('ref_axis',(0.,-3.01691039300315E-16,1.));
#28575=DIRECTION('center_axis',(0.,1.,3.01691039300315E-16));
#28576=DIRECTION('ref_axis',(0.,-3.01691039300315E-16,1.));
#28577=DIRECTION('',(0.,1.,3.01691039300315E-16));
#28578=DIRECTION('center_axis',(0.,1.,3.01691039300315E-16));
#28579=DIRECTION('ref_axis',(0.,-3.01691039300315E-16,1.));
#28580=DIRECTION('center_axis',(-1.,0.,0.));
#28581=DIRECTION('ref_axis',(0.,0.,1.));
#28582=DIRECTION('center_axis',(1.,0.,0.));
#28583=DIRECTION('ref_axis',(0.,0.,-1.));
#28584=DIRECTION('',(-1.,0.,0.));
#28585=DIRECTION('center_axis',(1.,0.,0.));
#28586=DIRECTION('ref_axis',(0.,0.,-1.));
#28587=DIRECTION('center_axis',(1.,0.,0.));
#28588=DIRECTION('ref_axis',(0.,0.,-1.));
#28589=DIRECTION('',(0.,-2.10269512239613E-16,1.));
#28590=DIRECTION('',(0.,-0.707106781186582,0.707106781186513));
#28591=DIRECTION('',(0.,-1.,-2.95272081017329E-16));
#28592=DIRECTION('',(0.,2.55331806268467E-16,-1.));
#28593=DIRECTION('',(0.,1.,5.90544162034659E-16));
#28594=DIRECTION('',(0.,0.707106781186562,0.707106781186533));
#28595=DIRECTION('',(0.,2.10269512239613E-16,1.));
#28596=DIRECTION('',(0.,1.,1.87537673078574E-16));
#28597=DIRECTION('',(0.,0.70710678118655,0.707106781186545));
#28598=DIRECTION('',(0.,0.,1.));
#28599=DIRECTION('',(0.,-0.707106781186543,0.707106781186552));
#28600=DIRECTION('',(0.,-1.,-7.50150692314296E-16));
#28601=DIRECTION('center_axis',(1.,0.,0.));
#28602=DIRECTION('ref_axis',(0.,0.,-1.));
#28603=DIRECTION('',(0.,-2.10269512239613E-16,1.));
#28604=DIRECTION('',(0.,-1.,-7.50150692314296E-16));
#28605=DIRECTION('',(0.,-0.707106781186543,0.707106781186552));
#28606=DIRECTION('',(0.,0.,1.));
#28607=DIRECTION('',(0.,0.70710678118655,0.707106781186545));
#28608=DIRECTION('',(0.,1.,1.87537673078574E-16));
#28609=DIRECTION('',(0.,2.10269512239613E-16,1.));
#28610=DIRECTION('',(0.,0.707106781186562,0.707106781186533));
#28611=DIRECTION('',(0.,1.,5.90544162034659E-16));
#28612=DIRECTION('',(0.,2.55331806268467E-16,-1.));
#28613=DIRECTION('',(0.,-1.,-2.95272081017329E-16));
#28614=DIRECTION('',(0.,-0.707106781186582,0.707106781186513));
#28615=DIRECTION('center_axis',(0.,-1.,-2.10269512239613E-16));
#28616=DIRECTION('ref_axis',(0.,2.10269512239613E-16,-1.));
#28617=DIRECTION('',(-1.,0.,0.));
#28618=DIRECTION('',(-1.,0.,0.));
#28619=DIRECTION('center_axis',(0.,-0.707106781186513,-0.707106781186582));
#28620=DIRECTION('ref_axis',(0.,0.707106781186582,-0.707106781186513));
#28621=DIRECTION('',(-1.,0.,0.));
#28622=DIRECTION('center_axis',(0.,2.95272081017329E-16,-1.));
#28623=DIRECTION('ref_axis',(0.,1.,2.95272081017329E-16));
#28624=DIRECTION('',(-1.,0.,0.));
#28625=DIRECTION('center_axis',(0.,1.,2.55331806268467E-16));
#28626=DIRECTION('ref_axis',(0.,-2.55331806268467E-16,1.));
#28627=DIRECTION('',(-1.,0.,0.));
#28628=DIRECTION('center_axis',(0.,-5.90544162034659E-16,1.));
#28629=DIRECTION('ref_axis',(0.,-1.,-5.90544162034659E-16));
#28630=DIRECTION('',(-1.,0.,0.));
#28631=DIRECTION('center_axis',(0.,-0.707106781186533,0.707106781186562));
#28632=DIRECTION('ref_axis',(0.,-0.707106781186562,-0.707106781186533));
#28633=DIRECTION('',(-1.,0.,0.));
#28634=DIRECTION('center_axis',(0.,-1.,2.10269512239613E-16));
#28635=DIRECTION('ref_axis',(0.,-2.10269512239613E-16,-1.));
#28636=DIRECTION('',(-1.,0.,0.));
#28637=DIRECTION('center_axis',(0.,-1.87537673078574E-16,1.));
#28638=DIRECTION('ref_axis',(0.,-1.,-1.87537673078574E-16));
#28639=DIRECTION('',(-1.,0.,0.));
#28640=DIRECTION('center_axis',(0.,-0.707106781186545,0.70710678118655));
#28641=DIRECTION('ref_axis',(0.,-0.70710678118655,-0.707106781186545));
#28642=DIRECTION('',(-1.,0.,0.));
#28643=DIRECTION('center_axis',(0.,-1.,0.));
#28644=DIRECTION('ref_axis',(0.,0.,-1.));
#28645=DIRECTION('',(-1.,0.,0.));
#28646=DIRECTION('center_axis',(0.,-0.707106781186552,-0.707106781186543));
#28647=DIRECTION('ref_axis',(0.,0.707106781186543,-0.707106781186553));
#28648=DIRECTION('',(-1.,0.,0.));
#28649=DIRECTION('center_axis',(0.,7.50150692314296E-16,-1.));
#28650=DIRECTION('ref_axis',(0.,1.,7.50150692314296E-16));
#28651=DIRECTION('center_axis',(-1.,-1.73472347597681E-16,0.));
#28652=DIRECTION('ref_axis',(3.17206578464331E-16,-1.,0.));
#28653=DIRECTION('center_axis',(-1.,-1.73472347597681E-16,0.));
#28654=DIRECTION('ref_axis',(1.73472347597681E-16,-1.,0.));
#28655=DIRECTION('center_axis',(2.12442355226077E-32,-1.22464679914735E-16,
-1.));
#28656=DIRECTION('ref_axis',(0.,1.,-1.22464679914735E-16));
#28657=DIRECTION('center_axis',(-1.,-1.73472347597681E-16,0.));
#28658=DIRECTION('ref_axis',(1.73472347597681E-16,-1.,0.));
#28659=DIRECTION('center_axis',(-1.,-1.73472347597681E-16,0.));
#28660=DIRECTION('ref_axis',(1.73472347597681E-16,-1.,0.));
#28661=DIRECTION('',(-1.,-1.73472347597681E-16,0.));
#28662=DIRECTION('center_axis',(-1.,-1.73472347597681E-16,0.));
#28663=DIRECTION('ref_axis',(1.73472347597681E-16,-1.,0.));
#28664=DIRECTION('center_axis',(-1.,-1.73472347597681E-16,0.));
#28665=DIRECTION('ref_axis',(1.58603289232165E-16,-1.,0.));
#28666=DIRECTION('center_axis',(2.12442355226077E-32,-1.22464679914735E-16,
-1.));
#28667=DIRECTION('ref_axis',(-1.98254111540206E-16,1.,-1.22464679914735E-16));
#28668=DIRECTION('center_axis',(-1.,-1.73472347597681E-16,0.));
#28669=DIRECTION('ref_axis',(1.73472347597681E-16,-1.,0.));
#28670=DIRECTION('center_axis',(-1.,-1.73472347597681E-16,0.));
#28671=DIRECTION('ref_axis',(1.73472347597681E-16,-1.,0.));
#28672=DIRECTION('center_axis',(-1.,-1.73472347597681E-16,0.));
#28673=DIRECTION('ref_axis',(1.73472347597681E-16,-1.,0.));
#28674=DIRECTION('',(1.,1.73472347597681E-16,0.));
#28675=DIRECTION('center_axis',(-1.,-1.73472347597681E-16,0.));
#28676=DIRECTION('ref_axis',(1.73472347597681E-16,-1.,0.));
#28677=DIRECTION('center_axis',(-1.,-1.73472347597681E-16,0.));
#28678=DIRECTION('ref_axis',(1.73472347597681E-16,-1.,0.));
#28679=DIRECTION('center_axis',(-1.,-1.73472347597681E-16,0.));
#28680=DIRECTION('ref_axis',(1.73472347597681E-16,-1.,0.));
#28681=DIRECTION('',(-1.,-1.73472347597681E-16,0.));
#28682=DIRECTION('center_axis',(-1.,-1.73472347597681E-16,0.));
#28683=DIRECTION('ref_axis',(1.73472347597681E-16,-1.,0.));
#28684=DIRECTION('center_axis',(-1.,-1.73472347597681E-16,0.));
#28685=DIRECTION('ref_axis',(1.36642833800019E-16,-1.,0.));
#28686=DIRECTION('center_axis',(-1.,-1.73472347597681E-16,0.));
#28687=DIRECTION('ref_axis',(1.73472347597681E-16,-1.,0.));
#28688=DIRECTION('center_axis',(2.12442355226077E-32,-1.22464679914735E-16,
-1.));
#28689=DIRECTION('ref_axis',(-1.70803542250024E-16,1.,-1.22464679914735E-16));
#28690=DIRECTION('center_axis',(-1.,-1.73472347597681E-16,0.));
#28691=DIRECTION('ref_axis',(1.73472347597681E-16,-1.,0.));
#28692=DIRECTION('center_axis',(-1.,-1.73472347597681E-16,0.));
#28693=DIRECTION('ref_axis',(1.73472347597681E-16,-1.,0.));
#28694=DIRECTION('',(1.,1.73472347597681E-16,0.));
#28695=DIRECTION('center_axis',(-1.,-1.73472347597681E-16,0.));
#28696=DIRECTION('ref_axis',(1.73472347597681E-16,-1.,0.));
#28697=DIRECTION('center_axis',(-1.,-1.73472347597681E-16,0.));
#28698=DIRECTION('ref_axis',(1.36642833800019E-16,-1.,0.));
#28699=DIRECTION('center_axis',(2.12442355226077E-32,-1.22464679914735E-16,
-1.));
#28700=DIRECTION('ref_axis',(-1.70803542250024E-16,1.,-1.22464679914735E-16));
#28701=DIRECTION('center_axis',(-1.,-1.73472347597681E-16,0.));
#28702=DIRECTION('ref_axis',(1.73472347597681E-16,-1.,0.));
#28703=DIRECTION('center_axis',(-1.,-1.73472347597681E-16,0.));
#28704=DIRECTION('ref_axis',(1.73472347597681E-16,-1.,0.));
#28705=DIRECTION('center_axis',(-1.,-1.73472347597681E-16,0.));
#28706=DIRECTION('ref_axis',(1.73472347597681E-16,-1.,0.));
#28707=DIRECTION('',(-1.,-1.73472347597681E-16,0.));
#28708=DIRECTION('center_axis',(-1.,-1.73472347597681E-16,0.));
#28709=DIRECTION('ref_axis',(1.73472347597681E-16,-1.,0.));
#28710=DIRECTION('center_axis',(-1.,-1.73472347597681E-16,0.));
#28711=DIRECTION('ref_axis',(1.73472347597681E-16,-1.,0.));
#28712=DIRECTION('center_axis',(-1.,-1.73472347597681E-16,0.));
#28713=DIRECTION('ref_axis',(1.73472347597681E-16,-1.,0.));
#28714=DIRECTION('',(1.,1.73472347597681E-16,0.));
#28715=DIRECTION('center_axis',(-1.,-1.73472347597681E-16,0.));
#28716=DIRECTION('ref_axis',(1.73472347597681E-16,-1.,0.));
#28717=DIRECTION('center_axis',(-1.,-1.73472347597681E-16,0.));
#28718=DIRECTION('ref_axis',(1.73472347597681E-16,-1.,0.));
#28719=DIRECTION('center_axis',(-1.,-1.73472347597681E-16,0.));
#28720=DIRECTION('ref_axis',(1.73472347597681E-16,-1.,0.));
#28721=DIRECTION('center_axis',(1.,1.73472347597681E-16,0.));
#28722=DIRECTION('ref_axis',(-1.73472347597681E-16,1.,0.));
#28723=DIRECTION('center_axis',(1.,1.73472347597681E-16,0.));
#28724=DIRECTION('ref_axis',(-1.73472347597681E-16,1.,0.));
#28725=DIRECTION('center_axis',(1.,1.73472347597681E-16,0.));
#28726=DIRECTION('ref_axis',(-1.73472347597681E-16,1.,0.));
#28727=DIRECTION('center_axis',(-1.,-1.73472347597681E-16,0.));
#28728=DIRECTION('ref_axis',(1.73472347597681E-16,-1.,0.));
#35877=CARTESIAN_POINT('',(0.,0.,0.));
#35878=CARTESIAN_POINT('Origin',(10.,24.,26.));
#35879=CARTESIAN_POINT('',(10.,-1.77635683940025E-14,21.5));
#35880=CARTESIAN_POINT('Origin',(10.,-1.73472347597681E-14,26.));
#35881=CARTESIAN_POINT('',(10.,24.,21.5));
#35882=CARTESIAN_POINT('',(10.,24.,21.5));
#35883=CARTESIAN_POINT('Origin',(10.,24.,26.));
#35884=CARTESIAN_POINT('Origin',(10.,24.,-26.));
#35885=CARTESIAN_POINT('',(10.,-4.44089209850063E-15,-30.5));
#35886=CARTESIAN_POINT('Origin',(10.,-3.46944695195361E-15,-26.));
#35887=CARTESIAN_POINT('',(10.,24.,-30.5));
#35888=CARTESIAN_POINT('',(10.,24.,-30.5));
#35889=CARTESIAN_POINT('Origin',(10.,24.,-26.));
#35890=CARTESIAN_POINT('Origin',(20.,25.,0.));
#35891=CARTESIAN_POINT('',(20.,25.,-13.));
#35892=CARTESIAN_POINT('Origin',(20.,25.,0.));
#35893=CARTESIAN_POINT('',(0.,25.,-13.));
#35894=CARTESIAN_POINT('',(20.,25.,-13.));
#35895=CARTESIAN_POINT('Origin',(0.,25.,0.));
#35896=CARTESIAN_POINT('Origin',(20.,0.,0.));
#35897=CARTESIAN_POINT('',(20.,24.,18.0000000000001));
#35898=CARTESIAN_POINT('',(20.,24.,34.5));
#35899=CARTESIAN_POINT('',(20.,24.,18.0000000000001));
#35900=CARTESIAN_POINT('',(20.,23.5,35.));
#35901=CARTESIAN_POINT('',(20.,24.,34.5));
#35902=CARTESIAN_POINT('',(20.,7.70371977754894E-31,35.));
#35903=CARTESIAN_POINT('',(20.,23.5,35.));
#35904=CARTESIAN_POINT('',(20.,1.78732264387927E-14,-35.));
#35905=CARTESIAN_POINT('',(20.,7.70371977754894E-31,35.));
#35906=CARTESIAN_POINT('',(20.,23.5,-35.));
#35907=CARTESIAN_POINT('',(20.,23.5,-35.));
#35908=CARTESIAN_POINT('',(20.,24.,-34.5));
#35909=CARTESIAN_POINT('',(20.,24.,-34.5));
#35910=CARTESIAN_POINT('',(20.,24.,-17.9999999999999));
#35911=CARTESIAN_POINT('',(20.,24.,-17.9999999999999));
#35912=CARTESIAN_POINT('',(20.,42.5,-17.9999999999999));
#35913=CARTESIAN_POINT('',(20.,42.5,-17.9999999999999));
#35914=CARTESIAN_POINT('',(20.,43.,-17.4999999999999));
#35915=CARTESIAN_POINT('',(20.,43.,-17.4999999999999));
#35916=CARTESIAN_POINT('',(20.,43.,17.5));
#35917=CARTESIAN_POINT('',(20.,43.,17.5));
#35918=CARTESIAN_POINT('',(20.,42.5,18.0000000000001));
#35919=CARTESIAN_POINT('',(20.,42.5,18.0000000000001));
#35920=CARTESIAN_POINT('',(20.,42.5,18.0000000000001));
#35921=CARTESIAN_POINT('Origin',(0.,0.,0.));
#35922=CARTESIAN_POINT('',(0.,24.,18.0000000000001));
#35923=CARTESIAN_POINT('',(0.,24.,34.5));
#35924=CARTESIAN_POINT('',(0.,24.,18.0000000000001));
#35925=CARTESIAN_POINT('',(0.,42.5,18.0000000000001));
#35926=CARTESIAN_POINT('',(0.,42.5,18.0000000000001));
#35927=CARTESIAN_POINT('',(0.,43.,17.5));
#35928=CARTESIAN_POINT('',(0.,42.5,18.0000000000001));
#35929=CARTESIAN_POINT('',(0.,43.,-17.4999999999999));
#35930=CARTESIAN_POINT('',(0.,43.,17.5));
#35931=CARTESIAN_POINT('',(0.,42.5,-17.9999999999999));
#35932=CARTESIAN_POINT('',(0.,43.,-17.4999999999999));
#35933=CARTESIAN_POINT('',(0.,24.,-17.9999999999999));
#35934=CARTESIAN_POINT('',(0.,42.5,-17.9999999999999));
#35935=CARTESIAN_POINT('',(0.,24.,-34.5));
#35936=CARTESIAN_POINT('',(0.,24.,-17.9999999999999));
#35937=CARTESIAN_POINT('',(0.,23.5,-35.));
#35938=CARTESIAN_POINT('',(0.,24.,-34.5));
#35939=CARTESIAN_POINT('',(0.,1.78732264387927E-14,-35.));
#35940=CARTESIAN_POINT('',(0.,23.5,-35.));
#35941=CARTESIAN_POINT('',(0.,7.70371977754894E-31,35.));
#35942=CARTESIAN_POINT('',(0.,7.70371977754894E-31,35.));
#35943=CARTESIAN_POINT('',(0.,23.5,35.));
#35944=CARTESIAN_POINT('',(0.,23.5,35.));
#35945=CARTESIAN_POINT('',(0.,24.,34.5));
#35946=CARTESIAN_POINT('Origin',(20.,24.,18.0000000000001));
#35947=CARTESIAN_POINT('',(20.,24.,34.5));
#35948=CARTESIAN_POINT('',(20.,24.,18.0000000000001));
#35949=CARTESIAN_POINT('Origin',(20.,24.,34.5));
#35950=CARTESIAN_POINT('',(20.,23.5,35.));
#35951=CARTESIAN_POINT('Origin',(20.,23.5,35.));
#35952=CARTESIAN_POINT('',(20.,7.70371977754894E-31,35.));
#35953=CARTESIAN_POINT('Origin',(20.,7.70371977754894E-31,35.));
#35954=CARTESIAN_POINT('',(20.,1.78732264387927E-14,-35.));
#35955=CARTESIAN_POINT('Origin',(20.,23.5,-35.));
#35956=CARTESIAN_POINT('',(20.,23.5,-35.));
#35957=CARTESIAN_POINT('Origin',(20.,24.,-34.5));
#35958=CARTESIAN_POINT('',(20.,24.,-34.5));
#35959=CARTESIAN_POINT('Origin',(20.,24.,-17.9999999999999));
#35960=CARTESIAN_POINT('',(20.,24.,-17.9999999999999));
#35961=CARTESIAN_POINT('Origin',(20.,42.5,-17.9999999999999));
#35962=CARTESIAN_POINT('',(20.,42.5,-17.9999999999999));
#35963=CARTESIAN_POINT('Origin',(20.,43.,-17.4999999999999));
#35964=CARTESIAN_POINT('',(20.,43.,-17.4999999999999));
#35965=CARTESIAN_POINT('Origin',(20.,43.,17.5));
#35966=CARTESIAN_POINT('',(20.,43.,17.5));
#35967=CARTESIAN_POINT('Origin',(20.,42.5,18.0000000000001));
#35968=CARTESIAN_POINT('',(20.,42.5,18.0000000000001));
#35969=CARTESIAN_POINT('Origin',(20.,42.5,18.0000000000001));
#35970=CARTESIAN_POINT('Origin',(13.7,25.,0.));
#35971=CARTESIAN_POINT('',(14.,30.3,-6.49062803548096E-16));
#35972=CARTESIAN_POINT('Origin',(14.,25.,0.));
#35973=CARTESIAN_POINT('',(13.7,30.,-6.12323399573676E-16));
#35974=CARTESIAN_POINT('Origin',(13.7,30.3,-6.49062803548097E-16));
#35975=CARTESIAN_POINT('Origin',(13.7,25.,0.));
#35976=CARTESIAN_POINT('Origin',(0.,25.,0.));
#35977=CARTESIAN_POINT('',(6.3,30.,-6.12323399573676E-16));
#35978=CARTESIAN_POINT('',(-8.67361737988403E-16,30.,-6.12323399573676E-16));
#35979=CARTESIAN_POINT('Origin',(6.3,25.,0.));
#35980=CARTESIAN_POINT('Origin',(6.3,25.,0.));
#35981=CARTESIAN_POINT('',(6.,30.3,-6.49062803548097E-16));
#35982=CARTESIAN_POINT('Origin',(6.3,30.3,-6.49062803548097E-16));
#35983=CARTESIAN_POINT('Origin',(6.,25.,0.));
#35984=CARTESIAN_POINT('Origin',(0.,25.,0.));
#35985=CARTESIAN_POINT('',(6.,31.7,-8.20513355428726E-16));
#35986=CARTESIAN_POINT('Origin',(6.,25.,0.));
#35987=CARTESIAN_POINT('',(6.45,31.7,-8.20513355428726E-16));
#35988=CARTESIAN_POINT('',(-1.16226472890446E-15,31.7,-8.20513355428726E-16));
#35989=CARTESIAN_POINT('Origin',(6.45,25.,0.));
#35990=CARTESIAN_POINT('Origin',(0.,25.,0.));
#35991=CARTESIAN_POINT('',(6.45,34.8,-1.20015386316441E-15));
#35992=CARTESIAN_POINT('Origin',(6.45,25.,0.));
#35993=CARTESIAN_POINT('',(6.,34.8,-1.20015386316441E-15));
#35994=CARTESIAN_POINT('',(-1.70002900645727E-15,34.8,-1.20015386316441E-15));
#35995=CARTESIAN_POINT('Origin',(6.,25.,0.));
#35996=CARTESIAN_POINT('Origin',(6.3,25.,0.));
#35997=CARTESIAN_POINT('',(6.,37.7,-1.55530143491714E-15));
#35998=CARTESIAN_POINT('Origin',(6.,25.,0.));
#35999=CARTESIAN_POINT('',(6.3,38.,-1.59204083889156E-15));
#36000=CARTESIAN_POINT('Origin',(6.3,37.7,-1.55530143491714E-15));
#36001=CARTESIAN_POINT('Origin',(6.3,25.,0.));
#36002=CARTESIAN_POINT('Origin',(0.,25.,0.));
#36003=CARTESIAN_POINT('',(13.7,38.,-1.59204083889156E-15));
#36004=CARTESIAN_POINT('',(-2.25514051876985E-15,38.,-1.59204083889156E-15));
#36005=CARTESIAN_POINT('Origin',(13.7,25.,0.));
#36006=CARTESIAN_POINT('Origin',(13.7,25.,0.));
#36007=CARTESIAN_POINT('',(14.,37.7,-1.55530143491714E-15));
#36008=CARTESIAN_POINT('Origin',(13.7,37.7,-1.55530143491714E-15));
#36009=CARTESIAN_POINT('Origin',(14.,25.,0.));
#36010=CARTESIAN_POINT('Origin',(0.,25.,0.));
#36011=CARTESIAN_POINT('',(14.,34.8,-1.20015386316441E-15));
#36012=CARTESIAN_POINT('Origin',(14.,25.,0.));
#36013=CARTESIAN_POINT('',(13.55,34.8,-1.20015386316441E-15));
#36014=CARTESIAN_POINT('',(-1.70002900645727E-15,34.8,-1.20015386316441E-15));
#36015=CARTESIAN_POINT('Origin',(13.55,25.,0.));
#36016=CARTESIAN_POINT('Origin',(0.,25.,0.));
#36017=CARTESIAN_POINT('',(13.55,31.7,-8.20513355428726E-16));
#36018=CARTESIAN_POINT('Origin',(13.55,25.,0.));
#36019=CARTESIAN_POINT('',(14.,31.7,-8.20513355428726E-16));
#36020=CARTESIAN_POINT('',(-1.16226472890446E-15,31.7,-8.20513355428726E-16));
#36021=CARTESIAN_POINT('Origin',(14.,25.,0.));
#36022=CARTESIAN_POINT('Origin',(13.55,31.7,0.));
#36023=CARTESIAN_POINT('Origin',(14.,34.8,0.));
#36024=CARTESIAN_POINT('Origin',(6.,37.7,0.));
#36025=CARTESIAN_POINT('Origin',(6.45,34.8,0.));
#36026=CARTESIAN_POINT('Origin',(6.,31.7,0.));
#36027=CARTESIAN_POINT('Origin',(14.,30.3,0.));
#57013=UNCERTAINTY_MEASURE_WITH_UNIT(LENGTH_MEASURE(0.01),#57080,
'DISTANCE_ACCURACY_VALUE',
'Maximum model space distance between geometric entities at asserted c
onnectivities');
#57040=UNCERTAINTY_MEASURE_WITH_UNIT(LENGTH_MEASURE(0.01),#57080,
'DISTANCE_ACCURACY_VALUE',
'Maximum model space distance between geometric entities at asserted c
onnectivities');
#57052=(
GEOMETRIC_REPRESENTATION_CONTEXT(3)
GLOBAL_UNCERTAINTY_ASSIGNED_CONTEXT((#57013))
GLOBAL_UNIT_ASSIGNED_CONTEXT((#57080,#57082,#57083))
REPRESENTATION_CONTEXT('','3D')
);
#57079=(
GEOMETRIC_REPRESENTATION_CONTEXT(3)
GLOBAL_UNCERTAINTY_ASSIGNED_CONTEXT((#57040))
GLOBAL_UNIT_ASSIGNED_CONTEXT((#57080,#57082,#57083))
REPRESENTATION_CONTEXT('','3D')
);
#57080=(
LENGTH_UNIT()
NAMED_UNIT(*)
SI_UNIT(.MILLI.,.METRE.)
);
#57082=(
NAMED_UNIT(*)
PLANE_ANGLE_UNIT()
SI_UNIT($,.RADIAN.)
);
#57083=(
NAMED_UNIT(*)
SI_UNIT($,.STERADIAN.)
SOLID_ANGLE_UNIT()
);
#57095=SHAPE_DEFINITION_REPRESENTATION(#57139,#57260);
#57139=PRODUCT_DEFINITION_SHAPE('',$,#57299);
#57260=SHAPE_REPRESENTATION('',(#25277),#57052);
#57287=PRODUCT_DEFINITION_CONTEXT('part definition',#57403,'design');
#57299=PRODUCT_DEFINITION('Fixed Bearing Housing',
'Fixed Bearing Housing',#57337,#57287);
#57337=PRODUCT_DEFINITION_FORMATION('',$,#57416);
#57403=APPLICATION_CONTEXT(
'Core Data for Automotive Mechanical Design Process');
#57404=PRODUCT_CONTEXT('part definition',#57403,'mechanical');
#57416=PRODUCT('Fixed Bearing Housing','Fixed Bearing Housing',$,(#57404));
#57444=PRESENTATION_STYLE_ASSIGNMENT((#57446));
#57446=SURFACE_STYLE_USAGE(.BOTH.,#57448);
#57448=SURFACE_SIDE_STYLE('',(#57450));
#57450=SURFACE_STYLE_FILL_AREA(#57452);
#57452=FILL_AREA_STYLE('Opaque(202,209,238)',(#57454));
#57454=FILL_AREA_STYLE_COLOUR('Opaque(202,209,238)',#57456);
#57456=COLOUR_RGB('Opaque(202,209,238)',0.792156862745098,0.819607843137255,
0.933333333333333);
ENDSEC;
END-ISO-10303-21;
